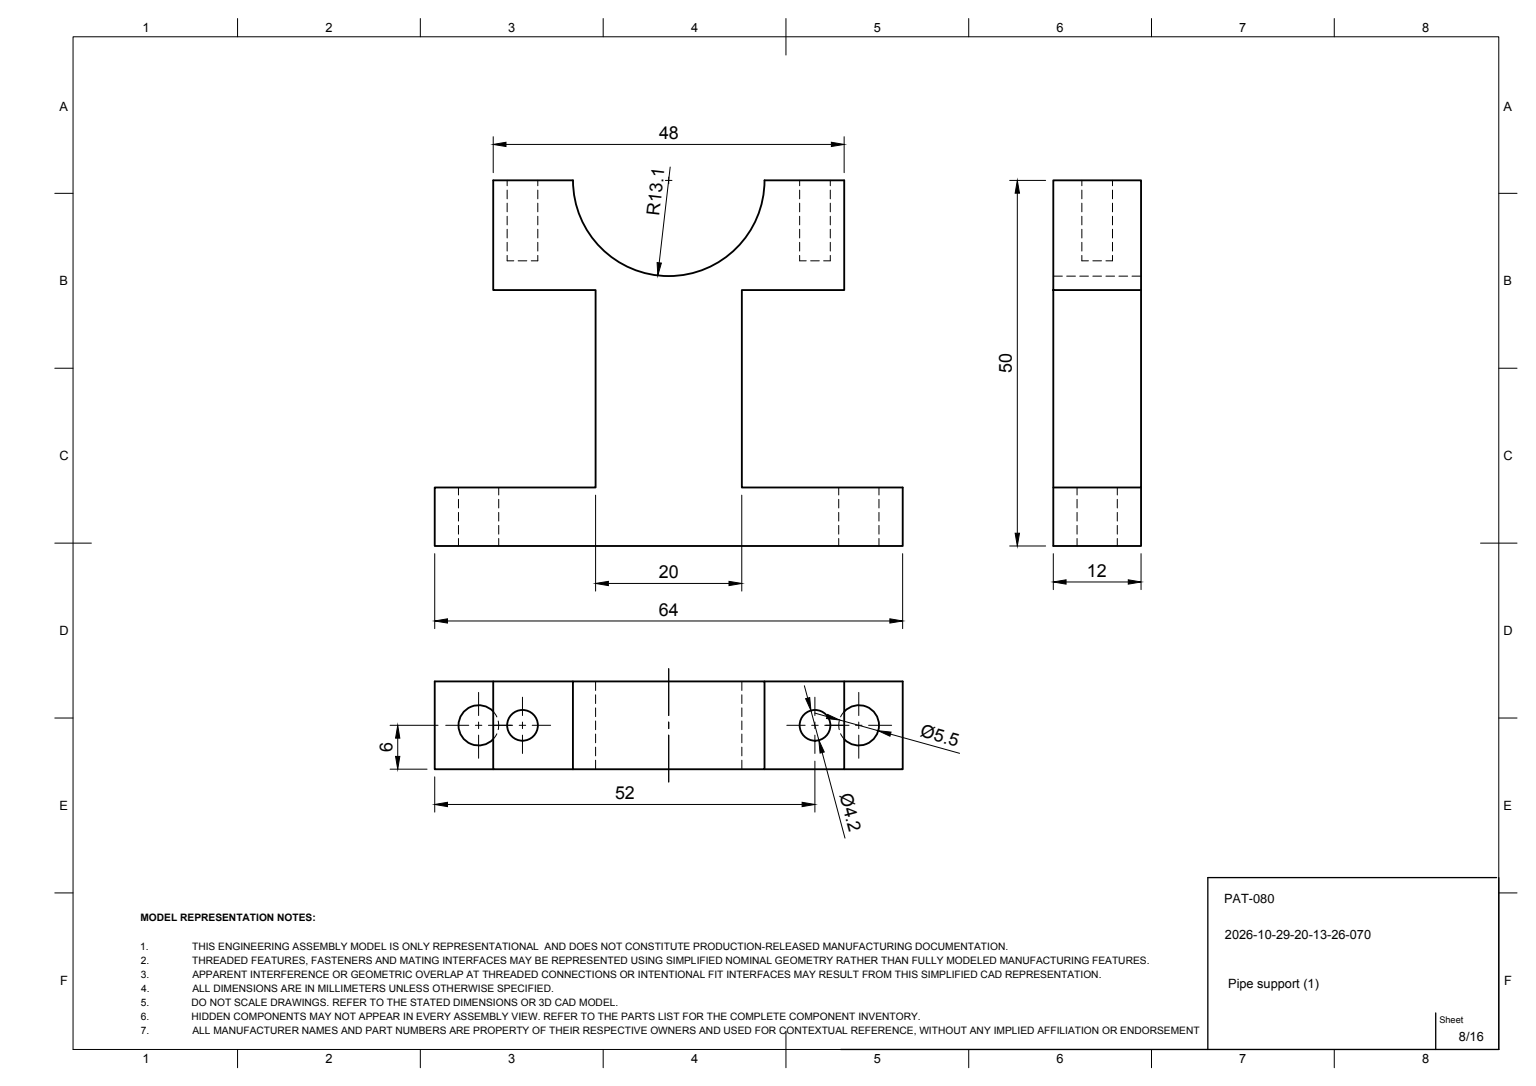
ISO-10303-21;
HEADER;
/* Generated by software containing ST-Developer
 * from STEP Tools, Inc. (www.steptools.com) 
 */

FILE_DESCRIPTION(
/* description */ ('PAT-080'),
/* implementation_level */ '2;1');

FILE_NAME(
/* name */ 'Pipe support (1).step',
/* time_stamp */ '2026-10-29T20:13:47-07:00',
/* author */ (''),
/* organization */ (''),
/* preprocessor_version */ 'ST-DEVELOPER v20.2',
/* originating_system */ 'Autodesk Translation Framework v15.17.0.0',
/* authorisation */ '');

FILE_SCHEMA (('AUTOMOTIVE_DESIGN { 1 0 10303 214 3 1 1 }'));
ENDSEC;

DATA;
#10=MECHANICAL_DESIGN_GEOMETRIC_PRESENTATION_REPRESENTATION('',(#251),#6878);
#213=SHAPE_REPRESENTATION_RELATIONSHIP('SRR','None',#6969,#232);
#232=ADVANCED_BREP_SHAPE_REPRESENTATION('',(#270),#6864);
#251=STYLED_ITEM('',(#7122),#270);
#270=MANIFOLD_SOLID_BREP('Body1',#3867);
#299=FACE_BOUND('',#811,.T.);
#300=FACE_BOUND('',#813,.T.);
#301=FACE_BOUND('',#815,.T.);
#302=FACE_BOUND('',#823,.T.);
#303=FACE_BOUND('',#826,.T.);
#304=FACE_BOUND('',#827,.T.);
#401=PLANE('',#4190);
#402=PLANE('',#4194);
#403=PLANE('',#4204);
#404=PLANE('',#4205);
#405=PLANE('',#4206);
#406=PLANE('',#4207);
#407=PLANE('',#4208);
#408=PLANE('',#4209);
#409=PLANE('',#4210);
#410=PLANE('',#4211);
#411=PLANE('',#4212);
#412=PLANE('',#4213);
#413=PLANE('',#4214);
#414=PLANE('',#4215);
#415=PLANE('',#4216);
#416=PLANE('',#4217);
#417=PLANE('',#4218);
#558=FACE_OUTER_BOUND('',#802,.T.);
#559=FACE_OUTER_BOUND('',#803,.T.);
#560=FACE_OUTER_BOUND('',#804,.T.);
#561=FACE_OUTER_BOUND('',#805,.T.);
#562=FACE_OUTER_BOUND('',#806,.T.);
#563=FACE_OUTER_BOUND('',#807,.T.);
#564=FACE_OUTER_BOUND('',#808,.T.);
#565=FACE_OUTER_BOUND('',#809,.T.);
#566=FACE_OUTER_BOUND('',#810,.T.);
#567=FACE_OUTER_BOUND('',#812,.T.);
#568=FACE_OUTER_BOUND('',#814,.T.);
#569=FACE_OUTER_BOUND('',#816,.T.);
#570=FACE_OUTER_BOUND('',#817,.T.);
#571=FACE_OUTER_BOUND('',#818,.T.);
#572=FACE_OUTER_BOUND('',#819,.T.);
#573=FACE_OUTER_BOUND('',#820,.T.);
#574=FACE_OUTER_BOUND('',#821,.T.);
#575=FACE_OUTER_BOUND('',#822,.T.);
#576=FACE_OUTER_BOUND('',#824,.T.);
#577=FACE_OUTER_BOUND('',#825,.T.);
#578=FACE_OUTER_BOUND('',#828,.T.);
#579=FACE_OUTER_BOUND('',#829,.T.);
#802=EDGE_LOOP('',(#2884,#2885,#2886,#2887));
#803=EDGE_LOOP('',(#2888));
#804=EDGE_LOOP('',(#2889,#2890,#2891,#2892));
#805=EDGE_LOOP('',(#2893));
#806=EDGE_LOOP('',(#2894,#2895,#2896,#2897));
#807=EDGE_LOOP('',(#2898,#2899,#2900,#2901));
#808=EDGE_LOOP('',(#2902,#2903,#2904,#2905));
#809=EDGE_LOOP('',(#2906,#2907,#2908,#2909,#2910,#2911,#2912,#2913,#2914,
#2915,#2916,#2917,#2918,#2919));
#810=EDGE_LOOP('',(#2920,#2921,#2922,#2923));
#811=EDGE_LOOP('',(#2924));
#812=EDGE_LOOP('',(#2925,#2926,#2927,#2928));
#813=EDGE_LOOP('',(#2929));
#814=EDGE_LOOP('',(#2930,#2931,#2932,#2933));
#815=EDGE_LOOP('',(#2934));
#816=EDGE_LOOP('',(#2935,#2936,#2937,#2938));
#817=EDGE_LOOP('',(#2939,#2940,#2941,#2942));
#818=EDGE_LOOP('',(#2943,#2944,#2945,#2946));
#819=EDGE_LOOP('',(#2947,#2948,#2949,#2950));
#820=EDGE_LOOP('',(#2951,#2952,#2953,#2954));
#821=EDGE_LOOP('',(#2955,#2956,#2957,#2958));
#822=EDGE_LOOP('',(#2959,#2960,#2961,#2962));
#823=EDGE_LOOP('',(#2963));
#824=EDGE_LOOP('',(#2964,#2965,#2966,#2967));
#825=EDGE_LOOP('',(#2968,#2969,#2970,#2971));
#826=EDGE_LOOP('',(#2972));
#827=EDGE_LOOP('',(#2973));
#828=EDGE_LOOP('',(#2974,#2975,#2976,#2977));
#829=EDGE_LOOP('',(#2978,#2979,#2980,#2981,#2982,#2983,#2984,#2985,#2986,
#2987,#2988,#2989,#2990,#2991));
#1138=LINE('',#6028,#1453);
#1139=LINE('',#6035,#1454);
#1140=LINE('',#6042,#1455);
#1141=LINE('',#6048,#1456);
#1142=LINE('',#6053,#1457);
#1143=LINE('',#6057,#1458);
#1144=LINE('',#6061,#1459);
#1145=LINE('',#6063,#1460);
#1146=LINE('',#6065,#1461);
#1147=LINE('',#6067,#1462);
#1148=LINE('',#6069,#1463);
#1149=LINE('',#6071,#1464);
#1150=LINE('',#6073,#1465);
#1151=LINE('',#6075,#1466);
#1152=LINE('',#6077,#1467);
#1153=LINE('',#6079,#1468);
#1154=LINE('',#6081,#1469);
#1155=LINE('',#6083,#1470);
#1156=LINE('',#6084,#1471);
#1157=LINE('',#6087,#1472);
#1158=LINE('',#6088,#1473);
#1159=LINE('',#6091,#1474);
#1160=LINE('',#6092,#1475);
#1161=LINE('',#6096,#1476);
#1162=LINE('',#6097,#1477);
#1163=LINE('',#6098,#1478);
#1164=LINE('',#6101,#1479);
#1165=LINE('',#6102,#1480);
#1166=LINE('',#6105,#1481);
#1167=LINE('',#6106,#1482);
#1168=LINE('',#6108,#1483);
#1169=LINE('',#6111,#1484);
#1170=LINE('',#6112,#1485);
#1171=LINE('',#6115,#1486);
#1172=LINE('',#6116,#1487);
#1173=LINE('',#6119,#1488);
#1174=LINE('',#6120,#1489);
#1175=LINE('',#6123,#1490);
#1176=LINE('',#6124,#1491);
#1177=LINE('',#6127,#1492);
#1178=LINE('',#6128,#1493);
#1179=LINE('',#6131,#1494);
#1180=LINE('',#6132,#1495);
#1181=LINE('',#6134,#1496);
#1453=VECTOR('',#4834,0.21);
#1454=VECTOR('',#4843,0.21);
#1455=VECTOR('',#4852,0.275);
#1456=VECTOR('',#4859,0.275);
#1457=VECTOR('',#4864,1.);
#1458=VECTOR('',#4867,1.);
#1459=VECTOR('',#4872,1.);
#1460=VECTOR('',#4873,1.);
#1461=VECTOR('',#4874,1.);
#1462=VECTOR('',#4875,1.);
#1463=VECTOR('',#4876,1.);
#1464=VECTOR('',#4877,1.);
#1465=VECTOR('',#4878,1.);
#1466=VECTOR('',#4879,1.);
#1467=VECTOR('',#4880,1.);
#1468=VECTOR('',#4881,1.);
#1469=VECTOR('',#4882,1.);
#1470=VECTOR('',#4883,1.);
#1471=VECTOR('',#4884,1.);
#1472=VECTOR('',#4887,1.);
#1473=VECTOR('',#4888,1.);
#1474=VECTOR('',#4891,1.);
#1475=VECTOR('',#4892,1.);
#1476=VECTOR('',#4895,1.);
#1477=VECTOR('',#4896,1.);
#1478=VECTOR('',#4897,1.);
#1479=VECTOR('',#4900,1.);
#1480=VECTOR('',#4901,1.);
#1481=VECTOR('',#4904,1.);
#1482=VECTOR('',#4905,1.);
#1483=VECTOR('',#4908,1.);
#1484=VECTOR('',#4911,1.);
#1485=VECTOR('',#4912,1.);
#1486=VECTOR('',#4915,1.);
#1487=VECTOR('',#4916,1.);
#1488=VECTOR('',#4919,1.);
#1489=VECTOR('',#4920,1.);
#1490=VECTOR('',#4923,1.);
#1491=VECTOR('',#4924,1.);
#1492=VECTOR('',#4927,1.);
#1493=VECTOR('',#4928,1.);
#1494=VECTOR('',#4931,1.);
#1495=VECTOR('',#4932,1.);
#1496=VECTOR('',#4935,1.);
#1686=CIRCLE('',#4188,0.21);
#1687=CIRCLE('',#4189,0.21);
#1688=CIRCLE('',#4192,0.21);
#1689=CIRCLE('',#4193,0.21);
#1690=CIRCLE('',#4196,0.275);
#1691=CIRCLE('',#4197,0.275);
#1692=CIRCLE('',#4199,0.275);
#1693=CIRCLE('',#4200,0.275);
#1694=CIRCLE('',#4202,1.31);
#1695=CIRCLE('',#4203,1.31);
#1902=VERTEX_POINT('',#6025);
#1903=VERTEX_POINT('',#6027);
#1904=VERTEX_POINT('',#6032);
#1905=VERTEX_POINT('',#6034);
#1906=VERTEX_POINT('',#6039);
#1907=VERTEX_POINT('',#6041);
#1908=VERTEX_POINT('',#6045);
#1909=VERTEX_POINT('',#6047);
#1910=VERTEX_POINT('',#6051);
#1911=VERTEX_POINT('',#6052);
#1912=VERTEX_POINT('',#6054);
#1913=VERTEX_POINT('',#6056);
#1914=VERTEX_POINT('',#6060);
#1915=VERTEX_POINT('',#6062);
#1916=VERTEX_POINT('',#6064);
#1917=VERTEX_POINT('',#6066);
#1918=VERTEX_POINT('',#6068);
#1919=VERTEX_POINT('',#6070);
#1920=VERTEX_POINT('',#6072);
#1921=VERTEX_POINT('',#6074);
#1922=VERTEX_POINT('',#6076);
#1923=VERTEX_POINT('',#6078);
#1924=VERTEX_POINT('',#6080);
#1925=VERTEX_POINT('',#6082);
#1926=VERTEX_POINT('',#6086);
#1927=VERTEX_POINT('',#6090);
#1928=VERTEX_POINT('',#6094);
#1929=VERTEX_POINT('',#6095);
#1930=VERTEX_POINT('',#6100);
#1931=VERTEX_POINT('',#6104);
#1932=VERTEX_POINT('',#6110);
#1933=VERTEX_POINT('',#6114);
#1934=VERTEX_POINT('',#6118);
#1935=VERTEX_POINT('',#6122);
#1936=VERTEX_POINT('',#6126);
#1937=VERTEX_POINT('',#6130);
#2265=EDGE_CURVE('',#1902,#1902,#1686,.T.);
#2266=EDGE_CURVE('',#1902,#1903,#1138,.T.);
#2267=EDGE_CURVE('',#1903,#1903,#1687,.T.);
#2268=EDGE_CURVE('',#1904,#1904,#1688,.T.);
#2269=EDGE_CURVE('',#1904,#1905,#1139,.T.);
#2270=EDGE_CURVE('',#1905,#1905,#1689,.T.);
#2271=EDGE_CURVE('',#1906,#1906,#1690,.T.);
#2272=EDGE_CURVE('',#1906,#1907,#1140,.T.);
#2273=EDGE_CURVE('',#1907,#1907,#1691,.T.);
#2274=EDGE_CURVE('',#1908,#1908,#1692,.T.);
#2275=EDGE_CURVE('',#1908,#1909,#1141,.T.);
#2276=EDGE_CURVE('',#1909,#1909,#1693,.T.);
#2277=EDGE_CURVE('',#1910,#1911,#1142,.T.);
#2278=EDGE_CURVE('',#1912,#1910,#1694,.T.);
#2279=EDGE_CURVE('',#1913,#1912,#1143,.T.);
#2280=EDGE_CURVE('',#1911,#1913,#1695,.T.);
#2281=EDGE_CURVE('',#1910,#1914,#1144,.T.);
#2282=EDGE_CURVE('',#1914,#1915,#1145,.T.);
#2283=EDGE_CURVE('',#1915,#1916,#1146,.T.);
#2284=EDGE_CURVE('',#1916,#1917,#1147,.T.);
#2285=EDGE_CURVE('',#1917,#1918,#1148,.T.);
#2286=EDGE_CURVE('',#1918,#1919,#1149,.T.);
#2287=EDGE_CURVE('',#1919,#1920,#1150,.T.);
#2288=EDGE_CURVE('',#1920,#1921,#1151,.T.);
#2289=EDGE_CURVE('',#1921,#1922,#1152,.T.);
#2290=EDGE_CURVE('',#1922,#1923,#1153,.T.);
#2291=EDGE_CURVE('',#1923,#1924,#1154,.T.);
#2292=EDGE_CURVE('',#1924,#1925,#1155,.T.);
#2293=EDGE_CURVE('',#1925,#1912,#1156,.T.);
#2294=EDGE_CURVE('',#1911,#1926,#1157,.T.);
#2295=EDGE_CURVE('',#1926,#1914,#1158,.T.);
#2296=EDGE_CURVE('',#1927,#1925,#1159,.T.);
#2297=EDGE_CURVE('',#1927,#1913,#1160,.T.);
#2298=EDGE_CURVE('',#1928,#1929,#1161,.T.);
#2299=EDGE_CURVE('',#1929,#1918,#1162,.T.);
#2300=EDGE_CURVE('',#1928,#1917,#1163,.T.);
#2301=EDGE_CURVE('',#1930,#1928,#1164,.T.);
#2302=EDGE_CURVE('',#1930,#1916,#1165,.T.);
#2303=EDGE_CURVE('',#1931,#1930,#1166,.T.);
#2304=EDGE_CURVE('',#1931,#1915,#1167,.T.);
#2305=EDGE_CURVE('',#1926,#1931,#1168,.T.);
#2306=EDGE_CURVE('',#1932,#1927,#1169,.T.);
#2307=EDGE_CURVE('',#1932,#1924,#1170,.T.);
#2308=EDGE_CURVE('',#1933,#1932,#1171,.T.);
#2309=EDGE_CURVE('',#1933,#1923,#1172,.T.);
#2310=EDGE_CURVE('',#1934,#1933,#1173,.T.);
#2311=EDGE_CURVE('',#1934,#1922,#1174,.T.);
#2312=EDGE_CURVE('',#1935,#1934,#1175,.T.);
#2313=EDGE_CURVE('',#1935,#1921,#1176,.T.);
#2314=EDGE_CURVE('',#1936,#1935,#1177,.T.);
#2315=EDGE_CURVE('',#1936,#1920,#1178,.T.);
#2316=EDGE_CURVE('',#1937,#1936,#1179,.T.);
#2317=EDGE_CURVE('',#1937,#1919,#1180,.T.);
#2318=EDGE_CURVE('',#1929,#1937,#1181,.T.);
#2884=ORIENTED_EDGE('',*,*,#2265,.F.);
#2885=ORIENTED_EDGE('',*,*,#2266,.T.);
#2886=ORIENTED_EDGE('',*,*,#2267,.F.);
#2887=ORIENTED_EDGE('',*,*,#2266,.F.);
#2888=ORIENTED_EDGE('',*,*,#2265,.T.);
#2889=ORIENTED_EDGE('',*,*,#2268,.F.);
#2890=ORIENTED_EDGE('',*,*,#2269,.T.);
#2891=ORIENTED_EDGE('',*,*,#2270,.F.);
#2892=ORIENTED_EDGE('',*,*,#2269,.F.);
#2893=ORIENTED_EDGE('',*,*,#2268,.T.);
#2894=ORIENTED_EDGE('',*,*,#2271,.F.);
#2895=ORIENTED_EDGE('',*,*,#2272,.T.);
#2896=ORIENTED_EDGE('',*,*,#2273,.F.);
#2897=ORIENTED_EDGE('',*,*,#2272,.F.);
#2898=ORIENTED_EDGE('',*,*,#2274,.F.);
#2899=ORIENTED_EDGE('',*,*,#2275,.T.);
#2900=ORIENTED_EDGE('',*,*,#2276,.F.);
#2901=ORIENTED_EDGE('',*,*,#2275,.F.);
#2902=ORIENTED_EDGE('',*,*,#2277,.F.);
#2903=ORIENTED_EDGE('',*,*,#2278,.F.);
#2904=ORIENTED_EDGE('',*,*,#2279,.F.);
#2905=ORIENTED_EDGE('',*,*,#2280,.F.);
#2906=ORIENTED_EDGE('',*,*,#2278,.T.);
#2907=ORIENTED_EDGE('',*,*,#2281,.T.);
#2908=ORIENTED_EDGE('',*,*,#2282,.T.);
#2909=ORIENTED_EDGE('',*,*,#2283,.T.);
#2910=ORIENTED_EDGE('',*,*,#2284,.T.);
#2911=ORIENTED_EDGE('',*,*,#2285,.T.);
#2912=ORIENTED_EDGE('',*,*,#2286,.T.);
#2913=ORIENTED_EDGE('',*,*,#2287,.T.);
#2914=ORIENTED_EDGE('',*,*,#2288,.T.);
#2915=ORIENTED_EDGE('',*,*,#2289,.T.);
#2916=ORIENTED_EDGE('',*,*,#2290,.T.);
#2917=ORIENTED_EDGE('',*,*,#2291,.T.);
#2918=ORIENTED_EDGE('',*,*,#2292,.T.);
#2919=ORIENTED_EDGE('',*,*,#2293,.T.);
#2920=ORIENTED_EDGE('',*,*,#2277,.T.);
#2921=ORIENTED_EDGE('',*,*,#2294,.T.);
#2922=ORIENTED_EDGE('',*,*,#2295,.T.);
#2923=ORIENTED_EDGE('',*,*,#2281,.F.);
#2924=ORIENTED_EDGE('',*,*,#2267,.T.);
#2925=ORIENTED_EDGE('',*,*,#2279,.T.);
#2926=ORIENTED_EDGE('',*,*,#2293,.F.);
#2927=ORIENTED_EDGE('',*,*,#2296,.F.);
#2928=ORIENTED_EDGE('',*,*,#2297,.T.);
#2929=ORIENTED_EDGE('',*,*,#2270,.T.);
#2930=ORIENTED_EDGE('',*,*,#2298,.T.);
#2931=ORIENTED_EDGE('',*,*,#2299,.T.);
#2932=ORIENTED_EDGE('',*,*,#2285,.F.);
#2933=ORIENTED_EDGE('',*,*,#2300,.F.);
#2934=ORIENTED_EDGE('',*,*,#2273,.T.);
#2935=ORIENTED_EDGE('',*,*,#2301,.T.);
#2936=ORIENTED_EDGE('',*,*,#2300,.T.);
#2937=ORIENTED_EDGE('',*,*,#2284,.F.);
#2938=ORIENTED_EDGE('',*,*,#2302,.F.);
#2939=ORIENTED_EDGE('',*,*,#2303,.T.);
#2940=ORIENTED_EDGE('',*,*,#2302,.T.);
#2941=ORIENTED_EDGE('',*,*,#2283,.F.);
#2942=ORIENTED_EDGE('',*,*,#2304,.F.);
#2943=ORIENTED_EDGE('',*,*,#2305,.T.);
#2944=ORIENTED_EDGE('',*,*,#2304,.T.);
#2945=ORIENTED_EDGE('',*,*,#2282,.F.);
#2946=ORIENTED_EDGE('',*,*,#2295,.F.);
#2947=ORIENTED_EDGE('',*,*,#2306,.T.);
#2948=ORIENTED_EDGE('',*,*,#2296,.T.);
#2949=ORIENTED_EDGE('',*,*,#2292,.F.);
#2950=ORIENTED_EDGE('',*,*,#2307,.F.);
#2951=ORIENTED_EDGE('',*,*,#2308,.T.);
#2952=ORIENTED_EDGE('',*,*,#2307,.T.);
#2953=ORIENTED_EDGE('',*,*,#2291,.F.);
#2954=ORIENTED_EDGE('',*,*,#2309,.F.);
#2955=ORIENTED_EDGE('',*,*,#2310,.T.);
#2956=ORIENTED_EDGE('',*,*,#2309,.T.);
#2957=ORIENTED_EDGE('',*,*,#2290,.F.);
#2958=ORIENTED_EDGE('',*,*,#2311,.F.);
#2959=ORIENTED_EDGE('',*,*,#2312,.T.);
#2960=ORIENTED_EDGE('',*,*,#2311,.T.);
#2961=ORIENTED_EDGE('',*,*,#2289,.F.);
#2962=ORIENTED_EDGE('',*,*,#2313,.F.);
#2963=ORIENTED_EDGE('',*,*,#2276,.T.);
#2964=ORIENTED_EDGE('',*,*,#2314,.T.);
#2965=ORIENTED_EDGE('',*,*,#2313,.T.);
#2966=ORIENTED_EDGE('',*,*,#2288,.F.);
#2967=ORIENTED_EDGE('',*,*,#2315,.F.);
#2968=ORIENTED_EDGE('',*,*,#2316,.T.);
#2969=ORIENTED_EDGE('',*,*,#2315,.T.);
#2970=ORIENTED_EDGE('',*,*,#2287,.F.);
#2971=ORIENTED_EDGE('',*,*,#2317,.F.);
#2972=ORIENTED_EDGE('',*,*,#2271,.T.);
#2973=ORIENTED_EDGE('',*,*,#2274,.T.);
#2974=ORIENTED_EDGE('',*,*,#2318,.T.);
#2975=ORIENTED_EDGE('',*,*,#2317,.T.);
#2976=ORIENTED_EDGE('',*,*,#2286,.F.);
#2977=ORIENTED_EDGE('',*,*,#2299,.F.);
#2978=ORIENTED_EDGE('',*,*,#2280,.T.);
#2979=ORIENTED_EDGE('',*,*,#2297,.F.);
#2980=ORIENTED_EDGE('',*,*,#2306,.F.);
#2981=ORIENTED_EDGE('',*,*,#2308,.F.);
#2982=ORIENTED_EDGE('',*,*,#2310,.F.);
#2983=ORIENTED_EDGE('',*,*,#2312,.F.);
#2984=ORIENTED_EDGE('',*,*,#2314,.F.);
#2985=ORIENTED_EDGE('',*,*,#2316,.F.);
#2986=ORIENTED_EDGE('',*,*,#2318,.F.);
#2987=ORIENTED_EDGE('',*,*,#2298,.F.);
#2988=ORIENTED_EDGE('',*,*,#2301,.F.);
#2989=ORIENTED_EDGE('',*,*,#2303,.F.);
#2990=ORIENTED_EDGE('',*,*,#2305,.F.);
#2991=ORIENTED_EDGE('',*,*,#2294,.F.);
#3584=CYLINDRICAL_SURFACE('',#4187,0.21);
#3585=CYLINDRICAL_SURFACE('',#4191,0.21);
#3586=CYLINDRICAL_SURFACE('',#4195,0.275);
#3587=CYLINDRICAL_SURFACE('',#4198,0.275);
#3588=CYLINDRICAL_SURFACE('',#4201,1.31);
#3694=ADVANCED_FACE('',(#558),#3584,.F.);
#3695=ADVANCED_FACE('',(#559),#401,.T.);
#3696=ADVANCED_FACE('',(#560),#3585,.F.);
#3697=ADVANCED_FACE('',(#561),#402,.T.);
#3698=ADVANCED_FACE('',(#562),#3586,.F.);
#3699=ADVANCED_FACE('',(#563),#3587,.F.);
#3700=ADVANCED_FACE('',(#564),#3588,.F.);
#3701=ADVANCED_FACE('',(#565),#403,.T.);
#3702=ADVANCED_FACE('',(#566,#299),#404,.T.);
#3703=ADVANCED_FACE('',(#567,#300),#405,.T.);
#3704=ADVANCED_FACE('',(#568,#301),#406,.T.);
#3705=ADVANCED_FACE('',(#569),#407,.T.);
#3706=ADVANCED_FACE('',(#570),#408,.T.);
#3707=ADVANCED_FACE('',(#571),#409,.T.);
#3708=ADVANCED_FACE('',(#572),#410,.T.);
#3709=ADVANCED_FACE('',(#573),#411,.T.);
#3710=ADVANCED_FACE('',(#574),#412,.T.);
#3711=ADVANCED_FACE('',(#575,#302),#413,.T.);
#3712=ADVANCED_FACE('',(#576),#414,.T.);
#3713=ADVANCED_FACE('',(#577,#303,#304),#415,.T.);
#3714=ADVANCED_FACE('',(#578),#416,.T.);
#3715=ADVANCED_FACE('',(#579),#417,.F.);
#3867=CLOSED_SHELL('',(#3694,#3695,#3696,#3697,#3698,#3699,#3700,#3701,
#3702,#3703,#3704,#3705,#3706,#3707,#3708,#3709,#3710,#3711,#3712,#3713,
#3714,#3715));
#4186=AXIS2_PLACEMENT_3D('',#6023,#4828,#4829);
#4187=AXIS2_PLACEMENT_3D('',#6024,#4830,#4831);
#4188=AXIS2_PLACEMENT_3D('',#6026,#4832,#4833);
#4189=AXIS2_PLACEMENT_3D('',#6029,#4835,#4836);
#4190=AXIS2_PLACEMENT_3D('',#6030,#4837,#4838);
#4191=AXIS2_PLACEMENT_3D('',#6031,#4839,#4840);
#4192=AXIS2_PLACEMENT_3D('',#6033,#4841,#4842);
#4193=AXIS2_PLACEMENT_3D('',#6036,#4844,#4845);
#4194=AXIS2_PLACEMENT_3D('',#6037,#4846,#4847);
#4195=AXIS2_PLACEMENT_3D('',#6038,#4848,#4849);
#4196=AXIS2_PLACEMENT_3D('',#6040,#4850,#4851);
#4197=AXIS2_PLACEMENT_3D('',#6043,#4853,#4854);
#4198=AXIS2_PLACEMENT_3D('',#6044,#4855,#4856);
#4199=AXIS2_PLACEMENT_3D('',#6046,#4857,#4858);
#4200=AXIS2_PLACEMENT_3D('',#6049,#4860,#4861);
#4201=AXIS2_PLACEMENT_3D('',#6050,#4862,#4863);
#4202=AXIS2_PLACEMENT_3D('',#6055,#4865,#4866);
#4203=AXIS2_PLACEMENT_3D('',#6058,#4868,#4869);
#4204=AXIS2_PLACEMENT_3D('',#6059,#4870,#4871);
#4205=AXIS2_PLACEMENT_3D('',#6085,#4885,#4886);
#4206=AXIS2_PLACEMENT_3D('',#6089,#4889,#4890);
#4207=AXIS2_PLACEMENT_3D('',#6093,#4893,#4894);
#4208=AXIS2_PLACEMENT_3D('',#6099,#4898,#4899);
#4209=AXIS2_PLACEMENT_3D('',#6103,#4902,#4903);
#4210=AXIS2_PLACEMENT_3D('',#6107,#4906,#4907);
#4211=AXIS2_PLACEMENT_3D('',#6109,#4909,#4910);
#4212=AXIS2_PLACEMENT_3D('',#6113,#4913,#4914);
#4213=AXIS2_PLACEMENT_3D('',#6117,#4917,#4918);
#4214=AXIS2_PLACEMENT_3D('',#6121,#4921,#4922);
#4215=AXIS2_PLACEMENT_3D('',#6125,#4925,#4926);
#4216=AXIS2_PLACEMENT_3D('',#6129,#4929,#4930);
#4217=AXIS2_PLACEMENT_3D('',#6133,#4933,#4934);
#4218=AXIS2_PLACEMENT_3D('',#6135,#4936,#4937);
#4828=DIRECTION('axis',(0.,0.,1.));
#4829=DIRECTION('refdir',(1.,0.,0.));
#4830=DIRECTION('center_axis',(0.,0.,1.));
#4831=DIRECTION('ref_axis',(1.,0.,0.));
#4832=DIRECTION('center_axis',(0.,0.,1.));
#4833=DIRECTION('ref_axis',(1.,0.,0.));
#4834=DIRECTION('',(0.,0.,1.));
#4835=DIRECTION('center_axis',(0.,0.,-1.));
#4836=DIRECTION('ref_axis',(1.,0.,0.));
#4837=DIRECTION('center_axis',(0.,0.,1.));
#4838=DIRECTION('ref_axis',(1.,0.,0.));
#4839=DIRECTION('center_axis',(0.,0.,1.));
#4840=DIRECTION('ref_axis',(1.,0.,0.));
#4841=DIRECTION('center_axis',(0.,0.,1.));
#4842=DIRECTION('ref_axis',(1.,0.,0.));
#4843=DIRECTION('',(0.,0.,1.));
#4844=DIRECTION('center_axis',(0.,0.,-1.));
#4845=DIRECTION('ref_axis',(1.,0.,0.));
#4846=DIRECTION('center_axis',(0.,0.,1.));
#4847=DIRECTION('ref_axis',(1.,0.,0.));
#4848=DIRECTION('center_axis',(0.,0.,1.));
#4849=DIRECTION('ref_axis',(1.,0.,0.));
#4850=DIRECTION('center_axis',(0.,0.,1.));
#4851=DIRECTION('ref_axis',(1.,0.,0.));
#4852=DIRECTION('',(0.,0.,1.));
#4853=DIRECTION('center_axis',(0.,0.,-1.));
#4854=DIRECTION('ref_axis',(1.,0.,0.));
#4855=DIRECTION('center_axis',(0.,0.,1.));
#4856=DIRECTION('ref_axis',(1.,0.,0.));
#4857=DIRECTION('center_axis',(0.,0.,1.));
#4858=DIRECTION('ref_axis',(1.,0.,0.));
#4859=DIRECTION('',(0.,0.,1.));
#4860=DIRECTION('center_axis',(0.,0.,-1.));
#4861=DIRECTION('ref_axis',(1.,0.,0.));
#4862=DIRECTION('center_axis',(1.,0.,0.));
#4863=DIRECTION('ref_axis',(0.,0.,-1.));
#4864=DIRECTION('',(-1.,0.,0.));
#4865=DIRECTION('center_axis',(-1.,0.,0.));
#4866=DIRECTION('ref_axis',(0.,0.,-1.));
#4867=DIRECTION('',(1.,0.,0.));
#4868=DIRECTION('center_axis',(1.,0.,0.));
#4869=DIRECTION('ref_axis',(0.,0.,-1.));
#4870=DIRECTION('center_axis',(1.,0.,0.));
#4871=DIRECTION('ref_axis',(0.,0.,-1.));
#4872=DIRECTION('',(0.,-1.,0.));
#4873=DIRECTION('',(0.,0.,-1.));
#4874=DIRECTION('',(0.,1.,0.));
#4875=DIRECTION('',(0.,0.,-1.));
#4876=DIRECTION('',(0.,-1.,0.));
#4877=DIRECTION('',(0.,0.,-1.));
#4878=DIRECTION('',(0.,1.,0.));
#4879=DIRECTION('',(0.,0.,1.));
#4880=DIRECTION('',(0.,-1.,0.));
#4881=DIRECTION('',(0.,0.,1.));
#4882=DIRECTION('',(0.,1.,0.));
#4883=DIRECTION('',(0.,0.,1.));
#4884=DIRECTION('',(0.,-1.,0.));
#4885=DIRECTION('center_axis',(0.,0.,1.));
#4886=DIRECTION('ref_axis',(0.,-1.,0.));
#4887=DIRECTION('',(0.,-1.,0.));
#4888=DIRECTION('',(1.,0.,0.));
#4889=DIRECTION('center_axis',(0.,0.,1.));
#4890=DIRECTION('ref_axis',(0.,-1.,0.));
#4891=DIRECTION('',(1.,0.,0.));
#4892=DIRECTION('',(0.,-1.,0.));
#4893=DIRECTION('center_axis',(0.,0.,1.));
#4894=DIRECTION('ref_axis',(0.,-1.,0.));
#4895=DIRECTION('',(0.,-1.,0.));
#4896=DIRECTION('',(1.,0.,0.));
#4897=DIRECTION('',(1.,0.,0.));
#4898=DIRECTION('center_axis',(0.,-1.,0.));
#4899=DIRECTION('ref_axis',(0.,0.,-1.));
#4900=DIRECTION('',(0.,0.,-1.));
#4901=DIRECTION('',(1.,0.,0.));
#4902=DIRECTION('center_axis',(0.,0.,-1.));
#4903=DIRECTION('ref_axis',(0.,1.,0.));
#4904=DIRECTION('',(0.,1.,0.));
#4905=DIRECTION('',(1.,0.,0.));
#4906=DIRECTION('center_axis',(0.,-1.,0.));
#4907=DIRECTION('ref_axis',(0.,0.,-1.));
#4908=DIRECTION('',(0.,0.,-1.));
#4909=DIRECTION('center_axis',(0.,1.,0.));
#4910=DIRECTION('ref_axis',(0.,0.,1.));
#4911=DIRECTION('',(0.,0.,1.));
#4912=DIRECTION('',(1.,0.,0.));
#4913=DIRECTION('center_axis',(0.,0.,-1.));
#4914=DIRECTION('ref_axis',(0.,1.,0.));
#4915=DIRECTION('',(0.,1.,0.));
#4916=DIRECTION('',(1.,0.,0.));
#4917=DIRECTION('center_axis',(0.,1.,0.));
#4918=DIRECTION('ref_axis',(0.,0.,1.));
#4919=DIRECTION('',(0.,0.,1.));
#4920=DIRECTION('',(1.,0.,0.));
#4921=DIRECTION('center_axis',(0.,0.,1.));
#4922=DIRECTION('ref_axis',(0.,-1.,0.));
#4923=DIRECTION('',(0.,-1.,0.));
#4924=DIRECTION('',(1.,0.,0.));
#4925=DIRECTION('center_axis',(0.,1.,0.));
#4926=DIRECTION('ref_axis',(0.,0.,1.));
#4927=DIRECTION('',(0.,0.,1.));
#4928=DIRECTION('',(1.,0.,0.));
#4929=DIRECTION('center_axis',(0.,0.,-1.));
#4930=DIRECTION('ref_axis',(0.,1.,0.));
#4931=DIRECTION('',(0.,1.,0.));
#4932=DIRECTION('',(1.,0.,0.));
#4933=DIRECTION('center_axis',(0.,-1.,0.));
#4934=DIRECTION('ref_axis',(0.,0.,-1.));
#4935=DIRECTION('',(0.,0.,-1.));
#4936=DIRECTION('center_axis',(1.,0.,0.));
#4937=DIRECTION('ref_axis',(0.,0.,-1.));
#6023=CARTESIAN_POINT('',(0.,0.,0.));
#6024=CARTESIAN_POINT('Origin',(4.5,-2.,4.9));
#6025=CARTESIAN_POINT('',(4.29,-2.,4.9));
#6026=CARTESIAN_POINT('Origin',(4.5,-2.,4.9));
#6027=CARTESIAN_POINT('',(4.29,-2.,6.));
#6028=CARTESIAN_POINT('',(4.29,-2.,4.9));
#6029=CARTESIAN_POINT('Origin',(4.5,-2.,6.));
#6030=CARTESIAN_POINT('Origin',(4.5,-2.,4.9));
#6031=CARTESIAN_POINT('Origin',(4.5,2.,4.9));
#6032=CARTESIAN_POINT('',(4.29,2.,4.9));
#6033=CARTESIAN_POINT('Origin',(4.5,2.,4.9));
#6034=CARTESIAN_POINT('',(4.29,2.,6.));
#6035=CARTESIAN_POINT('',(4.29,2.,4.9));
#6036=CARTESIAN_POINT('Origin',(4.5,2.,6.));
#6037=CARTESIAN_POINT('Origin',(4.5,2.,4.9));
#6038=CARTESIAN_POINT('Origin',(4.5,-2.6,0.9));
#6039=CARTESIAN_POINT('',(4.225,-2.6,1.));
#6040=CARTESIAN_POINT('Origin',(4.5,-2.6,1.));
#6041=CARTESIAN_POINT('',(4.225,-2.6,1.8));
#6042=CARTESIAN_POINT('',(4.225,-2.6,0.9));
#6043=CARTESIAN_POINT('Origin',(4.5,-2.6,1.8));
#6044=CARTESIAN_POINT('Origin',(4.5,2.6,0.9));
#6045=CARTESIAN_POINT('',(4.225,2.6,1.));
#6046=CARTESIAN_POINT('Origin',(4.5,2.6,1.));
#6047=CARTESIAN_POINT('',(4.225,2.6,1.8));
#6048=CARTESIAN_POINT('',(4.225,2.6,0.9));
#6049=CARTESIAN_POINT('Origin',(4.5,2.6,1.8));
#6050=CARTESIAN_POINT('Origin',(3.8,0.,6.));
#6051=CARTESIAN_POINT('',(5.1,-1.31,6.));
#6052=CARTESIAN_POINT('',(3.9,-1.31,6.));
#6053=CARTESIAN_POINT('',(3.8,-1.31,6.));
#6054=CARTESIAN_POINT('',(5.1,1.31,6.));
#6055=CARTESIAN_POINT('Origin',(5.1,0.,6.));
#6056=CARTESIAN_POINT('',(3.9,1.31,6.));
#6057=CARTESIAN_POINT('',(3.8,1.31,6.));
#6058=CARTESIAN_POINT('Origin',(3.9,0.,6.));
#6059=CARTESIAN_POINT('Origin',(5.1,0.,3.5));
#6060=CARTESIAN_POINT('',(5.1,-2.4,6.));
#6061=CARTESIAN_POINT('',(5.1,2.4,6.));
#6062=CARTESIAN_POINT('',(5.1,-2.4,4.5));
#6063=CARTESIAN_POINT('',(5.1,-2.4,6.));
#6064=CARTESIAN_POINT('',(5.1,-1.,4.5));
#6065=CARTESIAN_POINT('',(5.1,-2.4,4.5));
#6066=CARTESIAN_POINT('',(5.1,-1.,1.8));
#6067=CARTESIAN_POINT('',(5.1,-1.,4.5));
#6068=CARTESIAN_POINT('',(5.1,-3.2,1.8));
#6069=CARTESIAN_POINT('',(5.1,-1.,1.8));
#6070=CARTESIAN_POINT('',(5.1,-3.2,1.));
#6071=CARTESIAN_POINT('',(5.1,-3.2,1.8));
#6072=CARTESIAN_POINT('',(5.1,3.2,1.));
#6073=CARTESIAN_POINT('',(5.1,-3.2,1.));
#6074=CARTESIAN_POINT('',(5.1,3.2,1.8));
#6075=CARTESIAN_POINT('',(5.1,3.2,1.));
#6076=CARTESIAN_POINT('',(5.1,1.,1.8));
#6077=CARTESIAN_POINT('',(5.1,3.2,1.8));
#6078=CARTESIAN_POINT('',(5.1,1.,4.5));
#6079=CARTESIAN_POINT('',(5.1,1.,1.8));
#6080=CARTESIAN_POINT('',(5.1,2.4,4.5));
#6081=CARTESIAN_POINT('',(5.1,1.,4.5));
#6082=CARTESIAN_POINT('',(5.1,2.4,6.));
#6083=CARTESIAN_POINT('',(5.1,2.4,4.5));
#6084=CARTESIAN_POINT('',(5.1,2.4,6.));
#6085=CARTESIAN_POINT('Origin',(3.9,2.4,6.));
#6086=CARTESIAN_POINT('',(3.9,-2.4,6.));
#6087=CARTESIAN_POINT('',(3.9,2.4,6.));
#6088=CARTESIAN_POINT('',(3.9,-2.4,6.));
#6089=CARTESIAN_POINT('Origin',(3.9,2.4,6.));
#6090=CARTESIAN_POINT('',(3.9,2.4,6.));
#6091=CARTESIAN_POINT('',(3.9,2.4,6.));
#6092=CARTESIAN_POINT('',(3.9,2.4,6.));
#6093=CARTESIAN_POINT('Origin',(3.9,-1.,1.8));
#6094=CARTESIAN_POINT('',(3.9,-1.,1.8));
#6095=CARTESIAN_POINT('',(3.9,-3.2,1.8));
#6096=CARTESIAN_POINT('',(3.9,-1.,1.8));
#6097=CARTESIAN_POINT('',(3.9,-3.2,1.8));
#6098=CARTESIAN_POINT('',(3.9,-1.,1.8));
#6099=CARTESIAN_POINT('Origin',(3.9,-1.,4.5));
#6100=CARTESIAN_POINT('',(3.9,-1.,4.5));
#6101=CARTESIAN_POINT('',(3.9,-1.,4.5));
#6102=CARTESIAN_POINT('',(3.9,-1.,4.5));
#6103=CARTESIAN_POINT('Origin',(3.9,-2.4,4.5));
#6104=CARTESIAN_POINT('',(3.9,-2.4,4.5));
#6105=CARTESIAN_POINT('',(3.9,-2.4,4.5));
#6106=CARTESIAN_POINT('',(3.9,-2.4,4.5));
#6107=CARTESIAN_POINT('Origin',(3.9,-2.4,6.));
#6108=CARTESIAN_POINT('',(3.9,-2.4,6.));
#6109=CARTESIAN_POINT('Origin',(3.9,2.4,4.5));
#6110=CARTESIAN_POINT('',(3.9,2.4,4.5));
#6111=CARTESIAN_POINT('',(3.9,2.4,4.5));
#6112=CARTESIAN_POINT('',(3.9,2.4,4.5));
#6113=CARTESIAN_POINT('Origin',(3.9,1.,4.5));
#6114=CARTESIAN_POINT('',(3.9,1.,4.5));
#6115=CARTESIAN_POINT('',(3.9,1.,4.5));
#6116=CARTESIAN_POINT('',(3.9,1.,4.5));
#6117=CARTESIAN_POINT('Origin',(3.9,1.,1.8));
#6118=CARTESIAN_POINT('',(3.9,1.,1.8));
#6119=CARTESIAN_POINT('',(3.9,1.,1.8));
#6120=CARTESIAN_POINT('',(3.9,1.,1.8));
#6121=CARTESIAN_POINT('Origin',(3.9,3.2,1.8));
#6122=CARTESIAN_POINT('',(3.9,3.2,1.8));
#6123=CARTESIAN_POINT('',(3.9,3.2,1.8));
#6124=CARTESIAN_POINT('',(3.9,3.2,1.8));
#6125=CARTESIAN_POINT('Origin',(3.9,3.2,1.));
#6126=CARTESIAN_POINT('',(3.9,3.2,1.));
#6127=CARTESIAN_POINT('',(3.9,3.2,1.));
#6128=CARTESIAN_POINT('',(3.9,3.2,1.));
#6129=CARTESIAN_POINT('Origin',(3.9,-3.2,1.));
#6130=CARTESIAN_POINT('',(3.9,-3.2,1.));
#6131=CARTESIAN_POINT('',(3.9,-3.2,1.));
#6132=CARTESIAN_POINT('',(3.9,-3.2,1.));
#6133=CARTESIAN_POINT('Origin',(3.9,-3.2,1.8));
#6134=CARTESIAN_POINT('',(3.9,-3.2,1.8));
#6135=CARTESIAN_POINT('Origin',(3.9,0.,3.5));
#6843=UNCERTAINTY_MEASURE_WITH_UNIT(LENGTH_MEASURE(0.001),#6879,
'DISTANCE_ACCURACY_VALUE',
'Maximum model space distance between geometric entities at asserted c
onnectivities');
#6857=UNCERTAINTY_MEASURE_WITH_UNIT(LENGTH_MEASURE(0.001),#6879,
'DISTANCE_ACCURACY_VALUE',
'Maximum model space distance between geometric entities at asserted c
onnectivities');
#6864=(
GEOMETRIC_REPRESENTATION_CONTEXT(3)
GLOBAL_UNCERTAINTY_ASSIGNED_CONTEXT((#6843))
GLOBAL_UNIT_ASSIGNED_CONTEXT((#6879,#6881,#6882))
REPRESENTATION_CONTEXT('','3D')
);
#6878=(
GEOMETRIC_REPRESENTATION_CONTEXT(3)
GLOBAL_UNCERTAINTY_ASSIGNED_CONTEXT((#6857))
GLOBAL_UNIT_ASSIGNED_CONTEXT((#6879,#6881,#6882))
REPRESENTATION_CONTEXT('','3D')
);
#6879=(
LENGTH_UNIT()
NAMED_UNIT(*)
SI_UNIT(.CENTI.,.METRE.)
);
#6881=(
NAMED_UNIT(*)
PLANE_ANGLE_UNIT()
SI_UNIT($,.RADIAN.)
);
#6882=(
NAMED_UNIT(*)
SI_UNIT($,.STERADIAN.)
SOLID_ANGLE_UNIT()
);
#6889=SHAPE_DEFINITION_REPRESENTATION(#6909,#6969);
#6909=PRODUCT_DEFINITION_SHAPE('',$,#6990);
#6969=SHAPE_REPRESENTATION('',(#4186),#6864);
#6983=PRODUCT_DEFINITION_CONTEXT('part definition',#7045,'design');
#6990=PRODUCT_DEFINITION('Pipe support (1)','Pipe support (1)',#7010,
#6983);
#7010=PRODUCT_DEFINITION_FORMATION('',$,#7053);
#7045=APPLICATION_CONTEXT(
'Core Data for Automotive Mechanical Design Process');
#7046=PRODUCT_CONTEXT('part definition',#7045,'mechanical');
#7053=PRODUCT('Pipe support (1)','Pipe support (1)',
'Pipe support (1)',(#7046));
#7116=COLOUR_RGB('Sky Blue',0.24,0.69,0.87);
#7117=FILL_AREA_STYLE_COLOUR('',#7116);
#7118=FILL_AREA_STYLE('',(#7117));
#7119=SURFACE_STYLE_FILL_AREA(#7118);
#7120=SURFACE_SIDE_STYLE('',(#7119));
#7121=SURFACE_STYLE_USAGE(.BOTH.,#7120);
#7122=PRESENTATION_STYLE_ASSIGNMENT((#7121));
ENDSEC;
END-ISO-10303-21;
